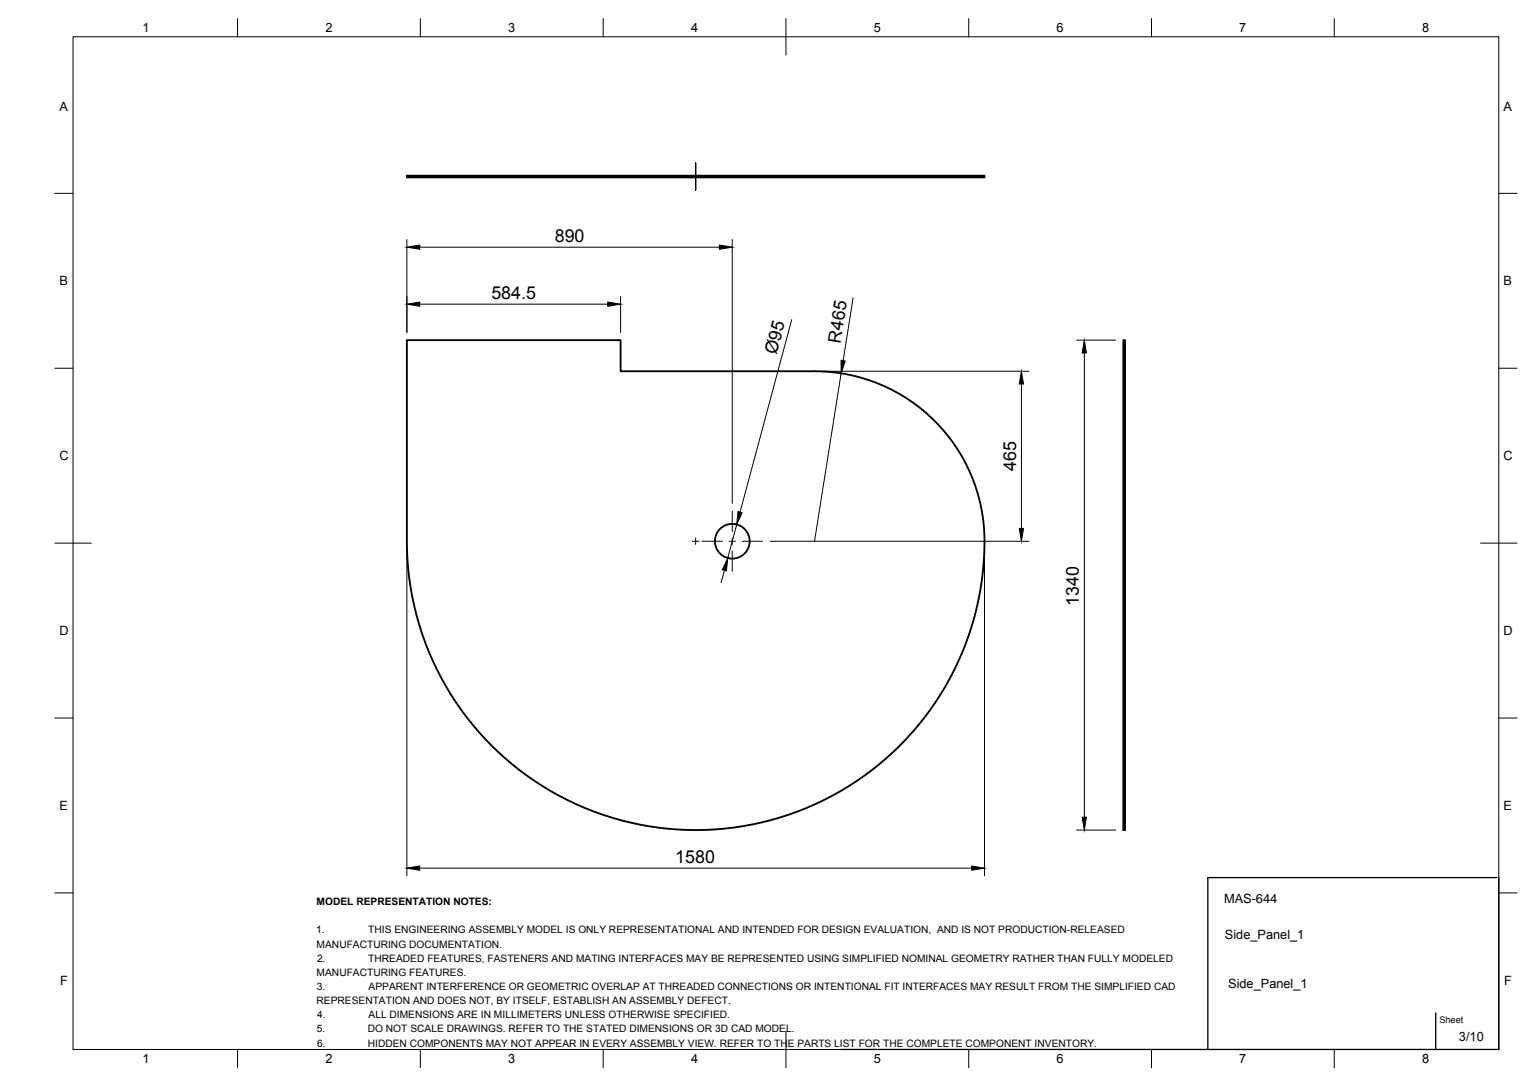
ISO-10303-21;
HEADER;
FILE_DESCRIPTION((''),'2;1');
FILE_NAME('Side_Panel_1.step','2026-10-09T11:38:21-07:00',(''),(''),'','','');
FILE_SCHEMA (('AUTOMOTIVE_DESIGN { 1 0 10303 214 3 1 1 }'));
ENDSEC;
DATA;
#10=MECHANICAL_DESIGN_GEOMETRIC_PRESENTATION_REPRESENTATION('',(#59),#3619);
#43=SHAPE_REPRESENTATION_RELATIONSHIP('SRR','None',#3651,#51) ;
#51=ADVANCED_BREP_SHAPE_REPRESENTATION('',(#67),#3611) ;
#59=STYLED_ITEM('',(#3700),#67) ;
#67=MANIFOLD_SOLID_BREP('Body1',#2083) ;
#75=FACE_BOUND('',#329,.T.) ;
#76=FACE_BOUND('',#331,.T.) ;
#157=PLANE('',#2185) ;
#158=PLANE('',#2186) ;
#159=PLANE('',#2187) ;
#160=PLANE('',#2188) ;
#161=PLANE('',#2195) ;
#162=PLANE('',#2196) ;
#213=FACE_OUTER_BOUND('',#321,.T.) ;
#214=FACE_OUTER_BOUND('',#322,.T.) ;
#215=FACE_OUTER_BOUND('',#323,.T.) ;
#216=FACE_OUTER_BOUND('',#324,.T.) ;
#217=FACE_OUTER_BOUND('',#325,.T.) ;
#218=FACE_OUTER_BOUND('',#326,.T.) ;
#219=FACE_OUTER_BOUND('',#327,.T.) ;
#220=FACE_OUTER_BOUND('',#328,.T.) ;
#221=FACE_OUTER_BOUND('',#330,.T.) ;
#321=EDGE_LOOP('',(#1387,#1388,#1389,#1390)) ;
#322=EDGE_LOOP('',(#1391,#1392,#1393,#1394)) ;
#323=EDGE_LOOP('',(#1395,#1396,#1397,#1398)) ;
#324=EDGE_LOOP('',(#1399,#1400,#1401,#1402)) ;
#325=EDGE_LOOP('',(#1403,#1404,#1405,#1406)) ;
#326=EDGE_LOOP('',(#1407,#1408,#1409,#1410)) ;
#327=EDGE_LOOP('',(#1411,#1412,#1413,#1414)) ;
#328=EDGE_LOOP('',(#1415,#1416,#1417,#1418,#1419,#1420)) ;
#329=EDGE_LOOP('',(#1421)) ;
#330=EDGE_LOOP('',(#1422,#1423,#1424,#1425,#1426,#1427)) ;
#331=EDGE_LOOP('',(#1428)) ;
#511=LINE('',#3037,#675) ;
#512=LINE('',#3042,#676) ;
#513=LINE('',#3044,#677) ;
#514=LINE('',#3046,#678) ;
#515=LINE('',#3047,#679) ;
#516=LINE('',#3050,#680) ;
#517=LINE('',#3052,#681) ;
#518=LINE('',#3053,#682) ;
#519=LINE('',#3056,#683) ;
#520=LINE('',#3058,#684) ;
#521=LINE('',#3059,#685) ;
#522=LINE('',#3062,#686) ;
#523=LINE('',#3064,#687) ;
#524=LINE('',#3065,#688) ;
#525=LINE('',#3070,#689) ;
#675=VECTOR('',#2417,47.5) ;
#676=VECTOR('',#2422,1000.) ;
#677=VECTOR('',#2423,1000.) ;
#678=VECTOR('',#2424,1000.) ;
#679=VECTOR('',#2425,1000.) ;
#680=VECTOR('',#2428,1000.) ;
#681=VECTOR('',#2429,1000.) ;
#682=VECTOR('',#2430,1000.) ;
#683=VECTOR('',#2433,1000.) ;
#684=VECTOR('',#2434,1000.) ;
#685=VECTOR('',#2435,1000.) ;
#686=VECTOR('',#2438,1000.) ;
#687=VECTOR('',#2439,1000.) ;
#688=VECTOR('',#2440,1000.) ;
#689=VECTOR('',#2445,1000.) ;
#839=CIRCLE('',#2183,47.5) ;
#840=CIRCLE('',#2184,47.5) ;
#841=CIRCLE('',#2190,790.) ;
#842=CIRCLE('',#2191,790.) ;
#843=CIRCLE('',#2193,465.) ;
#844=CIRCLE('',#2194,465.) ;
#943=VERTEX_POINT('',#3034) ;
#944=VERTEX_POINT('',#3036) ;
#945=VERTEX_POINT('',#3040) ;
#946=VERTEX_POINT('',#3041) ;
#947=VERTEX_POINT('',#3043) ;
#948=VERTEX_POINT('',#3045) ;
#949=VERTEX_POINT('',#3049) ;
#950=VERTEX_POINT('',#3051) ;
#951=VERTEX_POINT('',#3055) ;
#952=VERTEX_POINT('',#3057) ;
#953=VERTEX_POINT('',#3061) ;
#954=VERTEX_POINT('',#3063) ;
#955=VERTEX_POINT('',#3067) ;
#956=VERTEX_POINT('',#3069) ;
#1119=EDGE_CURVE('',#943,#943,#839,.T.) ;
#1120=EDGE_CURVE('',#943,#944,#511,.T.) ;
#1121=EDGE_CURVE('',#944,#944,#840,.T.) ;
#1122=EDGE_CURVE('',#945,#946,#512,.T.) ;
#1123=EDGE_CURVE('',#947,#945,#513,.T.) ;
#1124=EDGE_CURVE('',#947,#948,#514,.T.) ;
#1125=EDGE_CURVE('',#948,#946,#515,.T.) ;
#1126=EDGE_CURVE('',#949,#945,#516,.T.) ;
#1127=EDGE_CURVE('',#950,#949,#517,.T.) ;
#1128=EDGE_CURVE('',#950,#947,#518,.T.) ;
#1129=EDGE_CURVE('',#951,#949,#519,.T.) ;
#1130=EDGE_CURVE('',#952,#951,#520,.T.) ;
#1131=EDGE_CURVE('',#952,#950,#521,.T.) ;
#1132=EDGE_CURVE('',#953,#951,#522,.T.) ;
#1133=EDGE_CURVE('',#954,#953,#523,.T.) ;
#1134=EDGE_CURVE('',#954,#952,#524,.T.) ;
#1135=EDGE_CURVE('',#955,#953,#841,.T.) ;
#1136=EDGE_CURVE('',#956,#955,#525,.T.) ;
#1137=EDGE_CURVE('',#956,#954,#842,.T.) ;
#1138=EDGE_CURVE('',#946,#955,#843,.T.) ;
#1139=EDGE_CURVE('',#948,#956,#844,.T.) ;
#1387=ORIENTED_EDGE('',*,*,#1119,.F.) ;
#1388=ORIENTED_EDGE('',*,*,#1120,.T.) ;
#1389=ORIENTED_EDGE('',*,*,#1121,.T.) ;
#1390=ORIENTED_EDGE('',*,*,#1120,.F.) ;
#1391=ORIENTED_EDGE('',*,*,#1122,.F.) ;
#1392=ORIENTED_EDGE('',*,*,#1123,.F.) ;
#1393=ORIENTED_EDGE('',*,*,#1124,.T.) ;
#1394=ORIENTED_EDGE('',*,*,#1125,.T.) ;
#1395=ORIENTED_EDGE('',*,*,#1126,.F.) ;
#1396=ORIENTED_EDGE('',*,*,#1127,.F.) ;
#1397=ORIENTED_EDGE('',*,*,#1128,.T.) ;
#1398=ORIENTED_EDGE('',*,*,#1123,.T.) ;
#1399=ORIENTED_EDGE('',*,*,#1129,.F.) ;
#1400=ORIENTED_EDGE('',*,*,#1130,.F.) ;
#1401=ORIENTED_EDGE('',*,*,#1131,.T.) ;
#1402=ORIENTED_EDGE('',*,*,#1127,.T.) ;
#1403=ORIENTED_EDGE('',*,*,#1132,.F.) ;
#1404=ORIENTED_EDGE('',*,*,#1133,.F.) ;
#1405=ORIENTED_EDGE('',*,*,#1134,.T.) ;
#1406=ORIENTED_EDGE('',*,*,#1130,.T.) ;
#1407=ORIENTED_EDGE('',*,*,#1135,.F.) ;
#1408=ORIENTED_EDGE('',*,*,#1136,.F.) ;
#1409=ORIENTED_EDGE('',*,*,#1137,.T.) ;
#1410=ORIENTED_EDGE('',*,*,#1133,.T.) ;
#1411=ORIENTED_EDGE('',*,*,#1138,.F.) ;
#1412=ORIENTED_EDGE('',*,*,#1125,.F.) ;
#1413=ORIENTED_EDGE('',*,*,#1139,.T.) ;
#1414=ORIENTED_EDGE('',*,*,#1136,.T.) ;
#1415=ORIENTED_EDGE('',*,*,#1124,.F.) ;
#1416=ORIENTED_EDGE('',*,*,#1128,.F.) ;
#1417=ORIENTED_EDGE('',*,*,#1131,.F.) ;
#1418=ORIENTED_EDGE('',*,*,#1134,.F.) ;
#1419=ORIENTED_EDGE('',*,*,#1137,.F.) ;
#1420=ORIENTED_EDGE('',*,*,#1139,.F.) ;
#1421=ORIENTED_EDGE('',*,*,#1119,.T.) ;
#1422=ORIENTED_EDGE('',*,*,#1122,.T.) ;
#1423=ORIENTED_EDGE('',*,*,#1138,.T.) ;
#1424=ORIENTED_EDGE('',*,*,#1135,.T.) ;
#1425=ORIENTED_EDGE('',*,*,#1132,.T.) ;
#1426=ORIENTED_EDGE('',*,*,#1129,.T.) ;
#1427=ORIENTED_EDGE('',*,*,#1126,.T.) ;
#1428=ORIENTED_EDGE('',*,*,#1121,.F.) ;
#1923=CYLINDRICAL_SURFACE('',#2182,47.5) ;
#1924=CYLINDRICAL_SURFACE('',#2189,790.) ;
#1925=CYLINDRICAL_SURFACE('',#2192,465.) ;
#1975=ADVANCED_FACE('',(#213),#1923,.F.) ;
#1976=ADVANCED_FACE('',(#214),#157,.T.) ;
#1977=ADVANCED_FACE('',(#215),#158,.T.) ;
#1978=ADVANCED_FACE('',(#216),#159,.T.) ;
#1979=ADVANCED_FACE('',(#217),#160,.T.) ;
#1980=ADVANCED_FACE('',(#218),#1924,.T.) ;
#1981=ADVANCED_FACE('',(#219),#1925,.T.) ;
#1982=ADVANCED_FACE('',(#220,#75),#161,.T.) ;
#1983=ADVANCED_FACE('',(#221,#76),#162,.F.) ;
#2083=CLOSED_SHELL('',(#1975,#1976,#1977,#1978,#1979,#1980,#1981,#1982,
#1983)) ;
#2181=AXIS2_PLACEMENT_3D('',#3032,#2411,#2412) ;
#2182=AXIS2_PLACEMENT_3D('',#3033,#2413,#2414) ;
#2183=AXIS2_PLACEMENT_3D('',#3035,#2415,#2416) ;
#2184=AXIS2_PLACEMENT_3D('',#3038,#2418,#2419) ;
#2185=AXIS2_PLACEMENT_3D('',#3039,#2420,#2421) ;
#2186=AXIS2_PLACEMENT_3D('',#3048,#2426,#2427) ;
#2187=AXIS2_PLACEMENT_3D('',#3054,#2431,#2432) ;
#2188=AXIS2_PLACEMENT_3D('',#3060,#2436,#2437) ;
#2189=AXIS2_PLACEMENT_3D('',#3066,#2441,#2442) ;
#2190=AXIS2_PLACEMENT_3D('',#3068,#2443,#2444) ;
#2191=AXIS2_PLACEMENT_3D('',#3071,#2446,#2447) ;
#2192=AXIS2_PLACEMENT_3D('',#3072,#2448,#2449) ;
#2193=AXIS2_PLACEMENT_3D('',#3073,#2450,#2451) ;
#2194=AXIS2_PLACEMENT_3D('',#3074,#2452,#2453) ;
#2195=AXIS2_PLACEMENT_3D('',#3075,#2454,#2455) ;
#2196=AXIS2_PLACEMENT_3D('',#3076,#2456,#2457) ;
#2411=DIRECTION('axis',(0.,0.,1.)) ;
#2412=DIRECTION('refdir',(1.,0.,0.)) ;
#2413=DIRECTION('center_axis',(0.,0.,1.)) ;
#2414=DIRECTION('ref_axis',(1.,0.,0.)) ;
#2415=DIRECTION('center_axis',(0.,0.,1.)) ;
#2416=DIRECTION('ref_axis',(1.,0.,0.)) ;
#2417=DIRECTION('',(0.,0.,1.)) ;
#2418=DIRECTION('center_axis',(0.,0.,1.)) ;
#2419=DIRECTION('ref_axis',(1.,0.,0.)) ;
#2420=DIRECTION('center_axis',(1.81705896010664E-16,1.,0.)) ;
#2421=DIRECTION('ref_axis',(-1.,1.81705896010664E-16,0.)) ;
#2422=DIRECTION('',(-1.,1.81705896010664E-16,0.)) ;
#2423=DIRECTION('',(0.,0.,1.)) ;
#2424=DIRECTION('',(-1.,-2.46716227694479E-16,0.)) ;
#2425=DIRECTION('',(0.,0.,1.)) ;
#2426=DIRECTION('center_axis',(-1.,0.,0.)) ;
#2427=DIRECTION('ref_axis',(0.,0.,1.)) ;
#2428=DIRECTION('',(0.,-1.,0.)) ;
#2429=DIRECTION('',(0.,0.,1.)) ;
#2430=DIRECTION('',(0.,-1.,0.)) ;
#2431=DIRECTION('center_axis',(-1.89944058960677E-16,1.,0.)) ;
#2432=DIRECTION('ref_axis',(-1.,-1.89944058960677E-16,0.)) ;
#2433=DIRECTION('',(-1.,-1.89944058960677E-16,0.)) ;
#2434=DIRECTION('',(0.,0.,1.)) ;
#2435=DIRECTION('',(-1.,-1.89944058960677E-16,0.)) ;
#2436=DIRECTION('center_axis',(1.,0.,0.)) ;
#2437=DIRECTION('ref_axis',(0.,0.,-1.)) ;
#2438=DIRECTION('',(0.,1.,0.)) ;
#2439=DIRECTION('',(0.,0.,1.)) ;
#2440=DIRECTION('',(0.,1.,0.)) ;
#2441=DIRECTION('center_axis',(0.,0.,1.)) ;
#2442=DIRECTION('ref_axis',(1.,0.,0.)) ;
#2443=DIRECTION('center_axis',(0.,0.,1.)) ;
#2444=DIRECTION('ref_axis',(-1.,0.,0.)) ;
#2445=DIRECTION('',(0.,0.,1.)) ;
#2446=DIRECTION('center_axis',(0.,0.,1.)) ;
#2447=DIRECTION('ref_axis',(-1.,0.,0.)) ;
#2448=DIRECTION('center_axis',(0.,0.,1.)) ;
#2449=DIRECTION('ref_axis',(1.,0.,0.)) ;
#2450=DIRECTION('center_axis',(0.,0.,1.)) ;
#2451=DIRECTION('ref_axis',(-1.,0.,0.)) ;
#2452=DIRECTION('center_axis',(0.,0.,1.)) ;
#2453=DIRECTION('ref_axis',(-1.,0.,0.)) ;
#2454=DIRECTION('center_axis',(0.,0.,-1.)) ;
#2455=DIRECTION('ref_axis',(-1.,0.,0.)) ;
#2456=DIRECTION('center_axis',(0.,0.,-1.)) ;
#2457=DIRECTION('ref_axis',(-1.,0.,0.)) ;
#3032=CARTESIAN_POINT('',(0.,0.,0.)) ;
#3033=CARTESIAN_POINT('Origin',(0.,0.,-4.8)) ;
#3034=CARTESIAN_POINT('',(-47.5,-5.81707229594993E-15,-4.8)) ;
#3035=CARTESIAN_POINT('Origin',(0.,0.,-4.8)) ;
#3036=CARTESIAN_POINT('',(-47.5,-5.81707229594993E-15,0.)) ;
#3037=CARTESIAN_POINT('',(-47.5,-5.81707229594993E-15,-4.8)) ;
#3038=CARTESIAN_POINT('Origin',(0.,0.,0.)) ;
#3039=CARTESIAN_POINT('Origin',(0.,465.,-4.8)) ;
#3040=CARTESIAN_POINT('',(305.5,465.,0.)) ;
#3041=CARTESIAN_POINT('',(-225.,465.,0.)) ;
#3042=CARTESIAN_POINT('',(0.,465.,0.)) ;
#3043=CARTESIAN_POINT('',(305.5,465.,-4.8)) ;
#3044=CARTESIAN_POINT('',(305.5,465.,-4.8)) ;
#3045=CARTESIAN_POINT('',(-225.,465.,-4.8)) ;
#3046=CARTESIAN_POINT('',(-225.,465.,-4.8)) ;
#3047=CARTESIAN_POINT('',(-225.,465.,-4.8)) ;
#3048=CARTESIAN_POINT('Origin',(305.5,465.,-4.8)) ;
#3049=CARTESIAN_POINT('',(305.5,550.,0.)) ;
#3050=CARTESIAN_POINT('',(305.5,465.,0.)) ;
#3051=CARTESIAN_POINT('',(305.5,550.,-4.8)) ;
#3052=CARTESIAN_POINT('',(305.5,550.,-4.8)) ;
#3053=CARTESIAN_POINT('',(305.5,465.,-4.8)) ;
#3054=CARTESIAN_POINT('Origin',(305.5,550.,-4.8)) ;
#3055=CARTESIAN_POINT('',(890.,550.,0.)) ;
#3056=CARTESIAN_POINT('',(305.5,550.,0.)) ;
#3057=CARTESIAN_POINT('',(890.,550.,-4.8)) ;
#3058=CARTESIAN_POINT('',(890.,550.,-4.8)) ;
#3059=CARTESIAN_POINT('',(305.5,550.,-4.8)) ;
#3060=CARTESIAN_POINT('Origin',(890.,550.,-4.8)) ;
#3061=CARTESIAN_POINT('',(890.,-1.0683737973463E-15,0.)) ;
#3062=CARTESIAN_POINT('',(890.,550.,0.)) ;
#3063=CARTESIAN_POINT('',(890.,-1.0683737973463E-15,-4.8)) ;
#3064=CARTESIAN_POINT('',(890.,-1.0683737973463E-15,-4.8)) ;
#3065=CARTESIAN_POINT('',(890.,550.,-4.8)) ;
#3066=CARTESIAN_POINT('Origin',(100.,0.,-4.8)) ;
#3067=CARTESIAN_POINT('',(-690.,1.35308431126191E-13,0.)) ;
#3068=CARTESIAN_POINT('Origin',(100.,0.,0.)) ;
#3069=CARTESIAN_POINT('',(-690.,1.35308431126191E-13,-4.8)) ;
#3070=CARTESIAN_POINT('',(-690.,1.35308431126191E-13,-4.8)) ;
#3071=CARTESIAN_POINT('Origin',(100.,1.35308431126191E-13,-4.8)) ;
#3072=CARTESIAN_POINT('Origin',(-225.,1.35308431126191E-13,-4.8)) ;
#3073=CARTESIAN_POINT('Origin',(-225.,1.35308431126191E-13,0.)) ;
#3074=CARTESIAN_POINT('Origin',(-225.,1.35308431126191E-13,-4.8)) ;
#3075=CARTESIAN_POINT('Origin',(100.,0.,-4.8)) ;
#3076=CARTESIAN_POINT('Origin',(100.,0.,0.)) ;
#3601=UNCERTAINTY_MEASURE_WITH_UNIT(LENGTH_MEASURE(0.01),#3620,
'DISTANCE_ACCURACY_VALUE',
'Maximum model space distance between geometric entities at asserted c
onnectivities') ;
#3609=UNCERTAINTY_MEASURE_WITH_UNIT(LENGTH_MEASURE(0.01),#3620,
'DISTANCE_ACCURACY_VALUE',
'Maximum model space distance between geometric entities at asserted c
onnectivities') ;
#3611=(
GEOMETRIC_REPRESENTATION_CONTEXT(3)
GLOBAL_UNCERTAINTY_ASSIGNED_CONTEXT((#3601))
GLOBAL_UNIT_ASSIGNED_CONTEXT((#3620,#3622,#3623))
REPRESENTATION_CONTEXT('','3D')
) ;
#3619=(
GEOMETRIC_REPRESENTATION_CONTEXT(3)
GLOBAL_UNCERTAINTY_ASSIGNED_CONTEXT((#3609))
GLOBAL_UNIT_ASSIGNED_CONTEXT((#3620,#3622,#3623))
REPRESENTATION_CONTEXT('','3D')
) ;
#3620=(
LENGTH_UNIT()
NAMED_UNIT(*)
SI_UNIT(.MILLI.,.METRE.)
) ;
#3622=(
NAMED_UNIT(*)
PLANE_ANGLE_UNIT()
SI_UNIT($,.RADIAN.)
) ;
#3623=(
NAMED_UNIT(*)
SI_UNIT($,.STERADIAN.)
SOLID_ANGLE_UNIT()
) ;
#3625=SHAPE_DEFINITION_REPRESENTATION(#3634,#3651) ;
#3634=PRODUCT_DEFINITION_SHAPE('',$,#3661) ;
#3651=SHAPE_REPRESENTATION('',(#2181),#3611) ;
#3659=PRODUCT_DEFINITION_CONTEXT('part definition',#3688,'design') ;
#3661=PRODUCT_DEFINITION('Side_Panel_1','Side_Panel_1',#3670,#3659) ;
#3670=PRODUCT_DEFINITION_FORMATION('',$,#3691) ;
#3688=APPLICATION_CONTEXT(
'Core Data for Automotive Mechanical Design Process') ;
#3689=PRODUCT_CONTEXT('part definition',#3688,'mechanical') ;
#3691=PRODUCT('Side_Panel_1','Side_Panel_1',$,(#3689)) ;
#3700=PRESENTATION_STYLE_ASSIGNMENT((#3702)) ;
#3702=SURFACE_STYLE_USAGE(.BOTH.,#3704) ;
#3704=SURFACE_SIDE_STYLE('',(#3706)) ;
#3706=SURFACE_STYLE_FILL_AREA(#3708) ;
#3708=FILL_AREA_STYLE('Opaque(202,209,238)',(#3710)) ;
#3710=FILL_AREA_STYLE_COLOUR('Opaque(202,209,238)',#3712) ;
#3712=COLOUR_RGB('Opaque(202,209,238)', 0.09019608, 0.27058824, 0.51372549) ;
ENDSEC;
END-ISO-10303-21;
